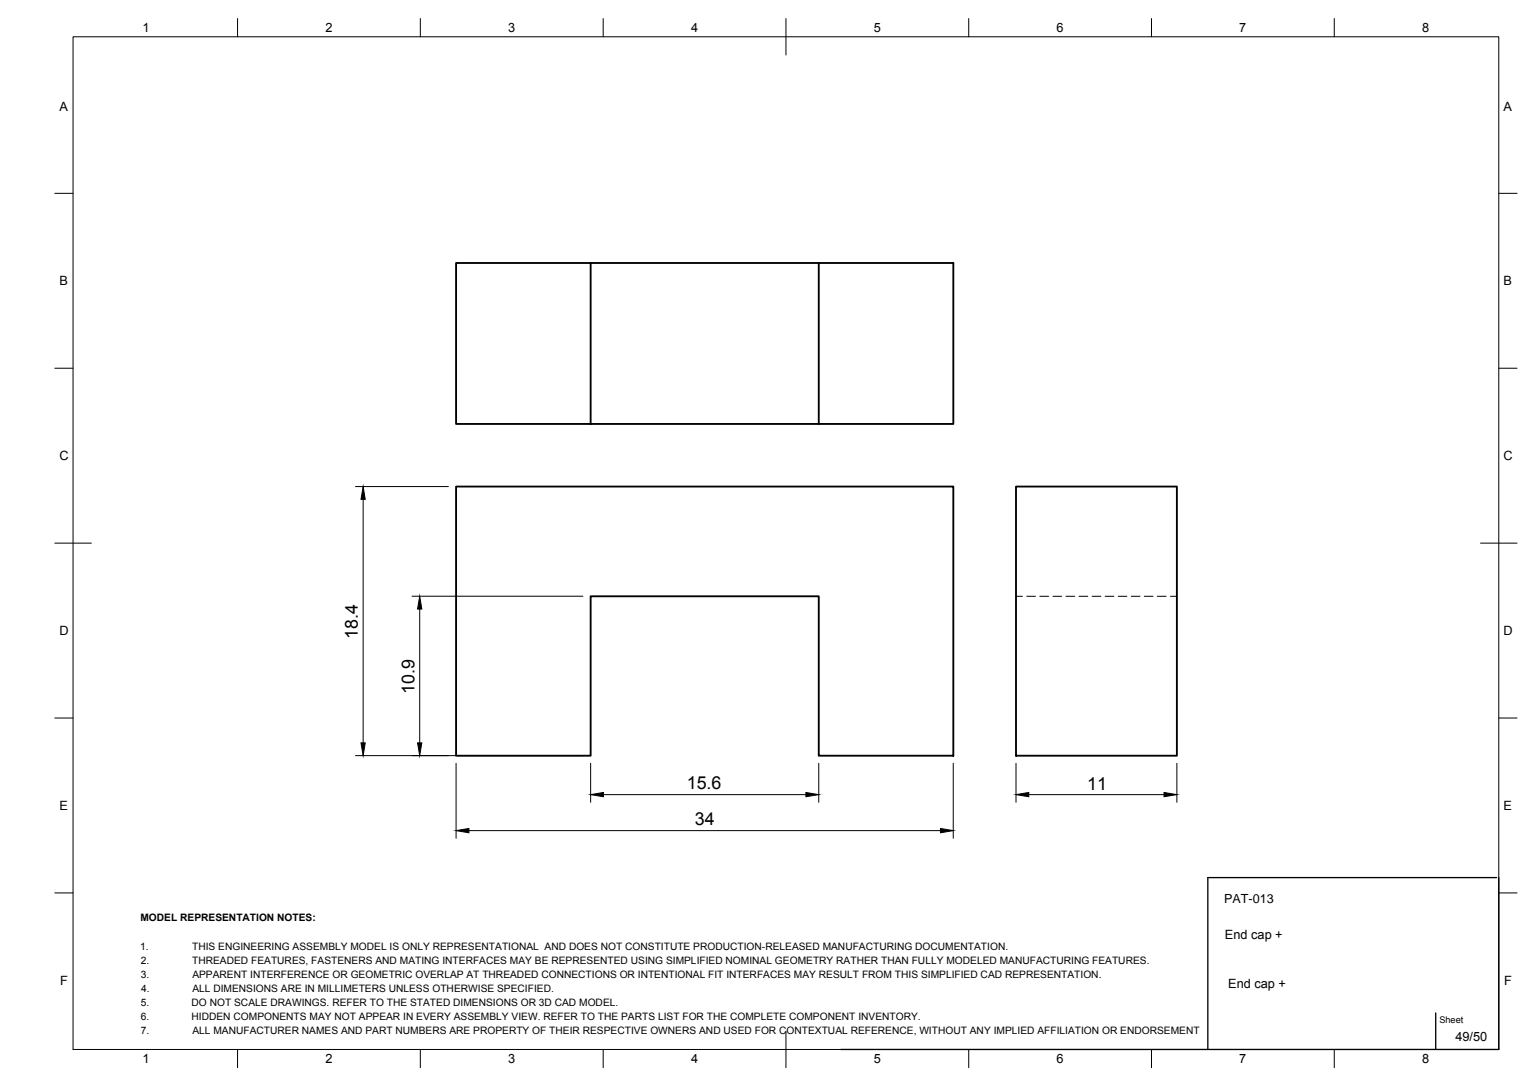
ISO-10303-21;
HEADER;
/* Generated by software containing ST-Developer
 * from STEP Tools, Inc. (www.steptools.com) 
 */

FILE_DESCRIPTION(
/* description */ ('Belt-driven linear axis on 2020 extrusion'),
/* implementation_level */ '2;1');

FILE_NAME(
/* name */ 'End cap +.step',
/* time_stamp */ '2026-10-28T03:26:09-07:00',
/* author */ (''),
/* organization */ (''),
/* preprocessor_version */ 'ST-DEVELOPER v20.2',
/* originating_system */ 'Autodesk Translation Framework v15.17.0.0',
/* authorisation */ '');

FILE_SCHEMA (('AUTOMOTIVE_DESIGN { 1 0 10303 214 3 1 1 }'));
ENDSEC;

DATA;
#10=MECHANICAL_DESIGN_GEOMETRIC_PRESENTATION_REPRESENTATION('',(#660),#20096);
#558=SHAPE_REPRESENTATION_RELATIONSHIP('SRR','None',#20359,#604);
#604=ADVANCED_BREP_SHAPE_REPRESENTATION('',(#715),#20090);
#660=STYLED_ITEM('',(#20643),#715);
#715=MANIFOLD_SOLID_BREP('Body1',#10974);
#1195=PLANE('',#12577);
#1196=PLANE('',#12578);
#1197=PLANE('',#12579);
#1198=PLANE('',#12580);
#1199=PLANE('',#12581);
#1200=PLANE('',#12582);
#1201=PLANE('',#12583);
#1202=PLANE('',#12584);
#1203=PLANE('',#12585);
#1204=PLANE('',#12586);
#1797=FACE_OUTER_BOUND('',#2585,.T.);
#1798=FACE_OUTER_BOUND('',#2586,.T.);
#1799=FACE_OUTER_BOUND('',#2587,.T.);
#1800=FACE_OUTER_BOUND('',#2588,.T.);
#1801=FACE_OUTER_BOUND('',#2589,.T.);
#1802=FACE_OUTER_BOUND('',#2590,.T.);
#1803=FACE_OUTER_BOUND('',#2591,.T.);
#1804=FACE_OUTER_BOUND('',#2592,.T.);
#1805=FACE_OUTER_BOUND('',#2593,.T.);
#1806=FACE_OUTER_BOUND('',#2594,.T.);
#2585=EDGE_LOOP('',(#9777,#9778,#9779,#9780));
#2586=EDGE_LOOP('',(#9781,#9782,#9783,#9784));
#2587=EDGE_LOOP('',(#9785,#9786,#9787,#9788));
#2588=EDGE_LOOP('',(#9789,#9790,#9791,#9792));
#2589=EDGE_LOOP('',(#9793,#9794,#9795,#9796));
#2590=EDGE_LOOP('',(#9797,#9798,#9799,#9800));
#2591=EDGE_LOOP('',(#9801,#9802,#9803,#9804));
#2592=EDGE_LOOP('',(#9805,#9806,#9807,#9808));
#2593=EDGE_LOOP('',(#9809,#9810,#9811,#9812,#9813,#9814,#9815,#9816));
#2594=EDGE_LOOP('',(#9817,#9818,#9819,#9820,#9821,#9822,#9823,#9824));
#3400=LINE('',#19566,#4257);
#3401=LINE('',#19568,#4258);
#3402=LINE('',#19570,#4259);
#3403=LINE('',#19571,#4260);
#3404=LINE('',#19574,#4261);
#3405=LINE('',#19576,#4262);
#3406=LINE('',#19577,#4263);
#3407=LINE('',#19580,#4264);
#3408=LINE('',#19582,#4265);
#3409=LINE('',#19583,#4266);
#3410=LINE('',#19586,#4267);
#3411=LINE('',#19588,#4268);
#3412=LINE('',#19589,#4269);
#3413=LINE('',#19592,#4270);
#3414=LINE('',#19594,#4271);
#3415=LINE('',#19595,#4272);
#3416=LINE('',#19598,#4273);
#3417=LINE('',#19600,#4274);
#3418=LINE('',#19601,#4275);
#3419=LINE('',#19604,#4276);
#3420=LINE('',#19606,#4277);
#3421=LINE('',#19607,#4278);
#3422=LINE('',#19609,#4279);
#3423=LINE('',#19610,#4280);
#4257=VECTOR('',#15696,1.);
#4258=VECTOR('',#15697,1.);
#4259=VECTOR('',#15698,1.);
#4260=VECTOR('',#15699,1.);
#4261=VECTOR('',#15702,1.);
#4262=VECTOR('',#15703,1.);
#4263=VECTOR('',#15704,1.);
#4264=VECTOR('',#15707,1.);
#4265=VECTOR('',#15708,1.);
#4266=VECTOR('',#15709,1.);
#4267=VECTOR('',#15712,1.);
#4268=VECTOR('',#15713,1.);
#4269=VECTOR('',#15714,1.);
#4270=VECTOR('',#15717,1.);
#4271=VECTOR('',#15718,1.);
#4272=VECTOR('',#15719,1.);
#4273=VECTOR('',#15722,1.);
#4274=VECTOR('',#15723,1.);
#4275=VECTOR('',#15724,1.);
#4276=VECTOR('',#15727,1.);
#4277=VECTOR('',#15728,1.);
#4278=VECTOR('',#15729,1.);
#4279=VECTOR('',#15732,1.);
#4280=VECTOR('',#15733,1.);
#5745=VERTEX_POINT('',#19564);
#5746=VERTEX_POINT('',#19565);
#5747=VERTEX_POINT('',#19567);
#5748=VERTEX_POINT('',#19569);
#5749=VERTEX_POINT('',#19573);
#5750=VERTEX_POINT('',#19575);
#5751=VERTEX_POINT('',#19579);
#5752=VERTEX_POINT('',#19581);
#5753=VERTEX_POINT('',#19585);
#5754=VERTEX_POINT('',#19587);
#5755=VERTEX_POINT('',#19591);
#5756=VERTEX_POINT('',#19593);
#5757=VERTEX_POINT('',#19597);
#5758=VERTEX_POINT('',#19599);
#5759=VERTEX_POINT('',#19603);
#5760=VERTEX_POINT('',#19605);
#7103=EDGE_CURVE('',#5745,#5746,#3400,.T.);
#7104=EDGE_CURVE('',#5746,#5747,#3401,.T.);
#7105=EDGE_CURVE('',#5748,#5747,#3402,.T.);
#7106=EDGE_CURVE('',#5745,#5748,#3403,.T.);
#7107=EDGE_CURVE('',#5749,#5745,#3404,.T.);
#7108=EDGE_CURVE('',#5750,#5748,#3405,.T.);
#7109=EDGE_CURVE('',#5749,#5750,#3406,.T.);
#7110=EDGE_CURVE('',#5751,#5749,#3407,.T.);
#7111=EDGE_CURVE('',#5752,#5750,#3408,.T.);
#7112=EDGE_CURVE('',#5751,#5752,#3409,.T.);
#7113=EDGE_CURVE('',#5753,#5751,#3410,.T.);
#7114=EDGE_CURVE('',#5754,#5752,#3411,.T.);
#7115=EDGE_CURVE('',#5753,#5754,#3412,.T.);
#7116=EDGE_CURVE('',#5755,#5753,#3413,.T.);
#7117=EDGE_CURVE('',#5756,#5754,#3414,.T.);
#7118=EDGE_CURVE('',#5755,#5756,#3415,.T.);
#7119=EDGE_CURVE('',#5757,#5755,#3416,.T.);
#7120=EDGE_CURVE('',#5758,#5756,#3417,.T.);
#7121=EDGE_CURVE('',#5757,#5758,#3418,.T.);
#7122=EDGE_CURVE('',#5759,#5757,#3419,.T.);
#7123=EDGE_CURVE('',#5760,#5758,#3420,.T.);
#7124=EDGE_CURVE('',#5759,#5760,#3421,.T.);
#7125=EDGE_CURVE('',#5746,#5759,#3422,.T.);
#7126=EDGE_CURVE('',#5747,#5760,#3423,.T.);
#9777=ORIENTED_EDGE('',*,*,#7103,.T.);
#9778=ORIENTED_EDGE('',*,*,#7104,.T.);
#9779=ORIENTED_EDGE('',*,*,#7105,.F.);
#9780=ORIENTED_EDGE('',*,*,#7106,.F.);
#9781=ORIENTED_EDGE('',*,*,#7107,.T.);
#9782=ORIENTED_EDGE('',*,*,#7106,.T.);
#9783=ORIENTED_EDGE('',*,*,#7108,.F.);
#9784=ORIENTED_EDGE('',*,*,#7109,.F.);
#9785=ORIENTED_EDGE('',*,*,#7110,.T.);
#9786=ORIENTED_EDGE('',*,*,#7109,.T.);
#9787=ORIENTED_EDGE('',*,*,#7111,.F.);
#9788=ORIENTED_EDGE('',*,*,#7112,.F.);
#9789=ORIENTED_EDGE('',*,*,#7113,.T.);
#9790=ORIENTED_EDGE('',*,*,#7112,.T.);
#9791=ORIENTED_EDGE('',*,*,#7114,.F.);
#9792=ORIENTED_EDGE('',*,*,#7115,.F.);
#9793=ORIENTED_EDGE('',*,*,#7116,.T.);
#9794=ORIENTED_EDGE('',*,*,#7115,.T.);
#9795=ORIENTED_EDGE('',*,*,#7117,.F.);
#9796=ORIENTED_EDGE('',*,*,#7118,.F.);
#9797=ORIENTED_EDGE('',*,*,#7119,.T.);
#9798=ORIENTED_EDGE('',*,*,#7118,.T.);
#9799=ORIENTED_EDGE('',*,*,#7120,.F.);
#9800=ORIENTED_EDGE('',*,*,#7121,.F.);
#9801=ORIENTED_EDGE('',*,*,#7122,.T.);
#9802=ORIENTED_EDGE('',*,*,#7121,.T.);
#9803=ORIENTED_EDGE('',*,*,#7123,.F.);
#9804=ORIENTED_EDGE('',*,*,#7124,.F.);
#9805=ORIENTED_EDGE('',*,*,#7125,.T.);
#9806=ORIENTED_EDGE('',*,*,#7124,.T.);
#9807=ORIENTED_EDGE('',*,*,#7126,.F.);
#9808=ORIENTED_EDGE('',*,*,#7104,.F.);
#9809=ORIENTED_EDGE('',*,*,#7126,.T.);
#9810=ORIENTED_EDGE('',*,*,#7123,.T.);
#9811=ORIENTED_EDGE('',*,*,#7120,.T.);
#9812=ORIENTED_EDGE('',*,*,#7117,.T.);
#9813=ORIENTED_EDGE('',*,*,#7114,.T.);
#9814=ORIENTED_EDGE('',*,*,#7111,.T.);
#9815=ORIENTED_EDGE('',*,*,#7108,.T.);
#9816=ORIENTED_EDGE('',*,*,#7105,.T.);
#9817=ORIENTED_EDGE('',*,*,#7125,.F.);
#9818=ORIENTED_EDGE('',*,*,#7103,.F.);
#9819=ORIENTED_EDGE('',*,*,#7107,.F.);
#9820=ORIENTED_EDGE('',*,*,#7110,.F.);
#9821=ORIENTED_EDGE('',*,*,#7113,.F.);
#9822=ORIENTED_EDGE('',*,*,#7116,.F.);
#9823=ORIENTED_EDGE('',*,*,#7119,.F.);
#9824=ORIENTED_EDGE('',*,*,#7122,.F.);
#10848=ADVANCED_FACE('',(#1797),#1195,.T.);
#10849=ADVANCED_FACE('',(#1798),#1196,.T.);
#10850=ADVANCED_FACE('',(#1799),#1197,.T.);
#10851=ADVANCED_FACE('',(#1800),#1198,.T.);
#10852=ADVANCED_FACE('',(#1801),#1199,.T.);
#10853=ADVANCED_FACE('',(#1802),#1200,.T.);
#10854=ADVANCED_FACE('',(#1803),#1201,.T.);
#10855=ADVANCED_FACE('',(#1804),#1202,.T.);
#10856=ADVANCED_FACE('',(#1805),#1203,.T.);
#10857=ADVANCED_FACE('',(#1806),#1204,.F.);
#10974=CLOSED_SHELL('',(#10848,#10849,#10850,#10851,#10852,#10853,#10854,
#10855,#10856,#10857));
#12576=AXIS2_PLACEMENT_3D('',#19562,#15692,#15693);
#12577=AXIS2_PLACEMENT_3D('',#19563,#15694,#15695);
#12578=AXIS2_PLACEMENT_3D('',#19572,#15700,#15701);
#12579=AXIS2_PLACEMENT_3D('',#19578,#15705,#15706);
#12580=AXIS2_PLACEMENT_3D('',#19584,#15710,#15711);
#12581=AXIS2_PLACEMENT_3D('',#19590,#15715,#15716);
#12582=AXIS2_PLACEMENT_3D('',#19596,#15720,#15721);
#12583=AXIS2_PLACEMENT_3D('',#19602,#15725,#15726);
#12584=AXIS2_PLACEMENT_3D('',#19608,#15730,#15731);
#12585=AXIS2_PLACEMENT_3D('',#19611,#15734,#15735);
#12586=AXIS2_PLACEMENT_3D('',#19612,#15736,#15737);
#15692=DIRECTION('axis',(0.,0.,1.));
#15693=DIRECTION('refdir',(1.,0.,0.));
#15694=DIRECTION('center_axis',(0.,0.,1.));
#15695=DIRECTION('ref_axis',(0.,-1.,0.));
#15696=DIRECTION('',(0.,-1.,0.));
#15697=DIRECTION('',(1.,0.,0.));
#15698=DIRECTION('',(0.,-1.,0.));
#15699=DIRECTION('',(1.,0.,0.));
#15700=DIRECTION('center_axis',(0.,1.,0.));
#15701=DIRECTION('ref_axis',(0.,0.,1.));
#15702=DIRECTION('',(0.,0.,1.));
#15703=DIRECTION('',(0.,0.,1.));
#15704=DIRECTION('',(1.,0.,0.));
#15705=DIRECTION('center_axis',(0.,0.,-1.));
#15706=DIRECTION('ref_axis',(0.,1.,0.));
#15707=DIRECTION('',(0.,1.,0.));
#15708=DIRECTION('',(0.,1.,0.));
#15709=DIRECTION('',(1.,0.,0.));
#15710=DIRECTION('center_axis',(0.,-1.,0.));
#15711=DIRECTION('ref_axis',(0.,0.,-1.));
#15712=DIRECTION('',(0.,0.,-1.));
#15713=DIRECTION('',(0.,0.,-1.));
#15714=DIRECTION('',(1.,0.,0.));
#15715=DIRECTION('center_axis',(0.,0.,-1.));
#15716=DIRECTION('ref_axis',(0.,1.,0.));
#15717=DIRECTION('',(0.,1.,0.));
#15718=DIRECTION('',(0.,1.,0.));
#15719=DIRECTION('',(1.,0.,0.));
#15720=DIRECTION('center_axis',(0.,1.,0.));
#15721=DIRECTION('ref_axis',(0.,0.,1.));
#15722=DIRECTION('',(0.,0.,1.));
#15723=DIRECTION('',(0.,0.,1.));
#15724=DIRECTION('',(1.,0.,0.));
#15725=DIRECTION('center_axis',(0.,0.,-1.));
#15726=DIRECTION('ref_axis',(0.,1.,0.));
#15727=DIRECTION('',(0.,1.,0.));
#15728=DIRECTION('',(0.,1.,0.));
#15729=DIRECTION('',(1.,0.,0.));
#15730=DIRECTION('center_axis',(0.,-1.,0.));
#15731=DIRECTION('ref_axis',(0.,0.,-1.));
#15732=DIRECTION('',(0.,0.,-1.));
#15733=DIRECTION('',(0.,0.,-1.));
#15734=DIRECTION('center_axis',(1.,0.,0.));
#15735=DIRECTION('ref_axis',(0.,0.,-1.));
#15736=DIRECTION('center_axis',(1.,0.,0.));
#15737=DIRECTION('ref_axis',(0.,0.,-1.));
#19562=CARTESIAN_POINT('',(0.,0.,0.));
#19563=CARTESIAN_POINT('Origin',(1.97,1.7,2.3));
#19564=CARTESIAN_POINT('',(1.97,1.7,2.3));
#19565=CARTESIAN_POINT('',(1.97,-1.7,2.3));
#19566=CARTESIAN_POINT('',(1.97,1.7,2.3));
#19567=CARTESIAN_POINT('',(3.07,-1.7,2.3));
#19568=CARTESIAN_POINT('',(1.97,-1.7,2.3));
#19569=CARTESIAN_POINT('',(3.07,1.7,2.3));
#19570=CARTESIAN_POINT('',(3.07,1.7,2.3));
#19571=CARTESIAN_POINT('',(1.97,1.7,2.3));
#19572=CARTESIAN_POINT('Origin',(1.97,1.7,0.46));
#19573=CARTESIAN_POINT('',(1.97,1.7,0.46));
#19574=CARTESIAN_POINT('',(1.97,1.7,0.46));
#19575=CARTESIAN_POINT('',(3.07,1.7,0.46));
#19576=CARTESIAN_POINT('',(3.07,1.7,0.46));
#19577=CARTESIAN_POINT('',(1.97,1.7,0.46));
#19578=CARTESIAN_POINT('Origin',(1.97,0.78,0.46));
#19579=CARTESIAN_POINT('',(1.97,0.78,0.46));
#19580=CARTESIAN_POINT('',(1.97,0.78,0.46));
#19581=CARTESIAN_POINT('',(3.07,0.78,0.46));
#19582=CARTESIAN_POINT('',(3.07,0.78,0.46));
#19583=CARTESIAN_POINT('',(1.97,0.78,0.46));
#19584=CARTESIAN_POINT('Origin',(1.97,0.78,1.55));
#19585=CARTESIAN_POINT('',(1.97,0.78,1.55));
#19586=CARTESIAN_POINT('',(1.97,0.78,1.55));
#19587=CARTESIAN_POINT('',(3.07,0.78,1.55));
#19588=CARTESIAN_POINT('',(3.07,0.78,1.55));
#19589=CARTESIAN_POINT('',(1.97,0.78,1.55));
#19590=CARTESIAN_POINT('Origin',(1.97,-0.78,1.55));
#19591=CARTESIAN_POINT('',(1.97,-0.78,1.55));
#19592=CARTESIAN_POINT('',(1.97,-0.78,1.55));
#19593=CARTESIAN_POINT('',(3.07,-0.78,1.55));
#19594=CARTESIAN_POINT('',(3.07,-0.78,1.55));
#19595=CARTESIAN_POINT('',(1.97,-0.78,1.55));
#19596=CARTESIAN_POINT('Origin',(1.97,-0.78,0.46));
#19597=CARTESIAN_POINT('',(1.97,-0.78,0.46));
#19598=CARTESIAN_POINT('',(1.97,-0.78,0.46));
#19599=CARTESIAN_POINT('',(3.07,-0.78,0.46));
#19600=CARTESIAN_POINT('',(3.07,-0.78,0.46));
#19601=CARTESIAN_POINT('',(1.97,-0.78,0.46));
#19602=CARTESIAN_POINT('Origin',(1.97,-1.7,0.46));
#19603=CARTESIAN_POINT('',(1.97,-1.7,0.46));
#19604=CARTESIAN_POINT('',(1.97,-1.7,0.46));
#19605=CARTESIAN_POINT('',(3.07,-1.7,0.46));
#19606=CARTESIAN_POINT('',(3.07,-1.7,0.46));
#19607=CARTESIAN_POINT('',(1.97,-1.7,0.46));
#19608=CARTESIAN_POINT('Origin',(1.97,-1.7,2.3));
#19609=CARTESIAN_POINT('',(1.97,-1.7,2.3));
#19610=CARTESIAN_POINT('',(3.07,-1.7,2.3));
#19611=CARTESIAN_POINT('Origin',(3.07,0.,1.38));
#19612=CARTESIAN_POINT('Origin',(1.97,0.,1.38));
#20036=UNCERTAINTY_MEASURE_WITH_UNIT(LENGTH_MEASURE(0.001),#20097,
'DISTANCE_ACCURACY_VALUE',
'Maximum model space distance between geometric entities at asserted c
onnectivities');
#20042=UNCERTAINTY_MEASURE_WITH_UNIT(LENGTH_MEASURE(0.001),#20097,
'DISTANCE_ACCURACY_VALUE',
'Maximum model space distance between geometric entities at asserted c
onnectivities');
#20090=(
GEOMETRIC_REPRESENTATION_CONTEXT(3)
GLOBAL_UNCERTAINTY_ASSIGNED_CONTEXT((#20036))
GLOBAL_UNIT_ASSIGNED_CONTEXT((#20097,#20099,#20100))
REPRESENTATION_CONTEXT('','3D')
);
#20096=(
GEOMETRIC_REPRESENTATION_CONTEXT(3)
GLOBAL_UNCERTAINTY_ASSIGNED_CONTEXT((#20042))
GLOBAL_UNIT_ASSIGNED_CONTEXT((#20097,#20099,#20100))
REPRESENTATION_CONTEXT('','3D')
);
#20097=(
LENGTH_UNIT()
NAMED_UNIT(*)
SI_UNIT(.CENTI.,.METRE.)
);
#20099=(
NAMED_UNIT(*)
PLANE_ANGLE_UNIT()
SI_UNIT($,.RADIAN.)
);
#20100=(
NAMED_UNIT(*)
SI_UNIT($,.STERADIAN.)
SOLID_ANGLE_UNIT()
);
#20148=SHAPE_DEFINITION_REPRESENTATION(#20206,#20359);
#20206=PRODUCT_DEFINITION_SHAPE('',$,#20413);
#20359=SHAPE_REPRESENTATION('',(#12576),#20090);
#20365=PRODUCT_DEFINITION_CONTEXT('part definition',#20526,'design');
#20413=PRODUCT_DEFINITION('End cap +','End cap +',#20466,#20365);
#20466=PRODUCT_DEFINITION_FORMATION('',$,#20575);
#20526=APPLICATION_CONTEXT(
'Core Data for Automotive Mechanical Design Process');
#20527=PRODUCT_CONTEXT('part definition',#20526,'mechanical');
#20575=PRODUCT('End cap +','End cap +','End cap +',(#20527));
#20637=COLOUR_RGB('Sky Blue',0.24,0.69,0.87);
#20638=FILL_AREA_STYLE_COLOUR('',#20637);
#20639=FILL_AREA_STYLE('',(#20638));
#20640=SURFACE_STYLE_FILL_AREA(#20639);
#20641=SURFACE_SIDE_STYLE('',(#20640));
#20642=SURFACE_STYLE_USAGE(.BOTH.,#20641);
#20643=PRESENTATION_STYLE_ASSIGNMENT((#20642));
ENDSEC;
END-ISO-10303-21;
